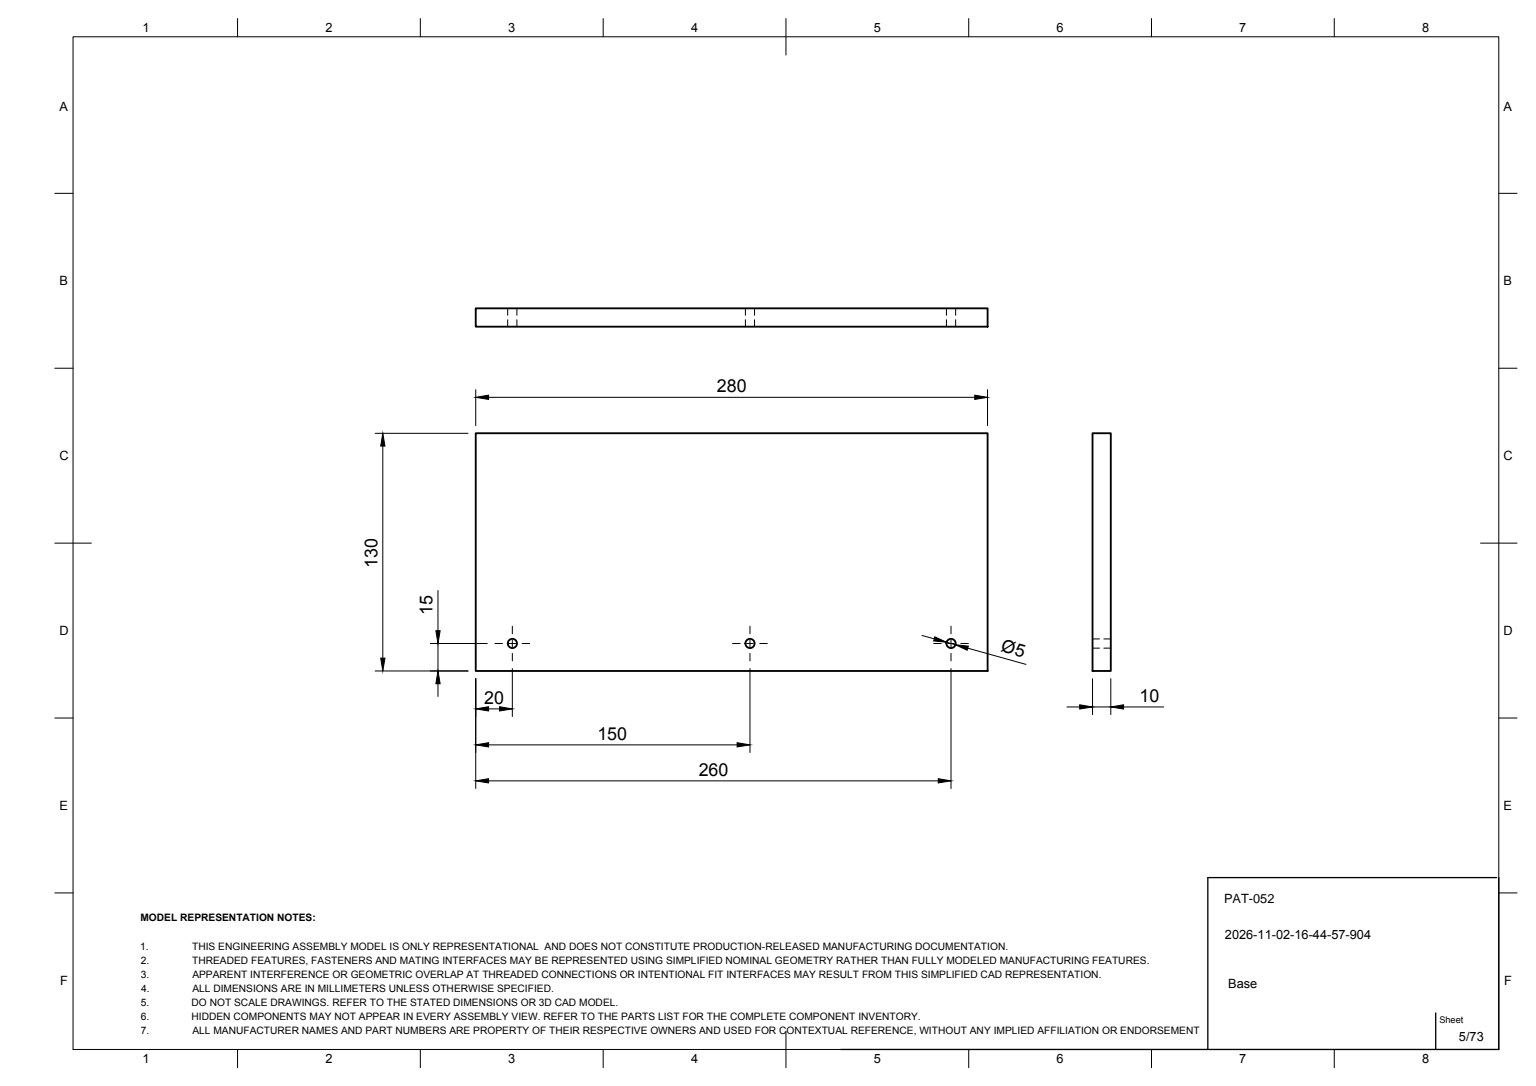
ISO-10303-21;
HEADER;
/* Generated by software containing ST-Developer
 * from STEP Tools, Inc. (www.steptools.com) 
 */

FILE_DESCRIPTION(
/* description */ ('Hand-crank gear train demonstrator'),
/* implementation_level */ '2;1');

FILE_NAME(
/* name */ 'Base.step',
/* time_stamp */ '2026-10-28T03:22:13-07:00',
/* author */ (''),
/* organization */ (''),
/* preprocessor_version */ 'ST-DEVELOPER v20.2',
/* originating_system */ 'Autodesk Translation Framework v15.17.0.0',
/* authorisation */ '');

FILE_SCHEMA (('AUTOMOTIVE_DESIGN { 1 0 10303 214 3 1 1 }'));
ENDSEC;

DATA;
#10=MECHANICAL_DESIGN_GEOMETRIC_PRESENTATION_REPRESENTATION('',(#1189),#62758);
#1061=SHAPE_REPRESENTATION_RELATIONSHIP('SRR','None',#63033,#1125);
#1125=ADVANCED_BREP_SHAPE_REPRESENTATION('',(#1268),#62687);
#1189=STYLED_ITEM('',(#63441),#1268);
#1268=MANIFOLD_SOLID_BREP('Body1',#16369);
#1342=FACE_BOUND('',#3067,.T.);
#1343=FACE_BOUND('',#3068,.T.);
#1344=FACE_BOUND('',#3069,.T.);
#1345=FACE_BOUND('',#3071,.T.);
#1346=FACE_BOUND('',#3072,.T.);
#1347=FACE_BOUND('',#3073,.T.);
#1633=PLANE('',#17170);
#1634=PLANE('',#17171);
#1635=PLANE('',#17172);
#1636=PLANE('',#17173);
#1637=PLANE('',#17174);
#1638=PLANE('',#17175);
#2123=FACE_OUTER_BOUND('',#3059,.T.);
#2124=FACE_OUTER_BOUND('',#3060,.T.);
#2125=FACE_OUTER_BOUND('',#3061,.T.);
#2126=FACE_OUTER_BOUND('',#3062,.T.);
#2127=FACE_OUTER_BOUND('',#3063,.T.);
#2128=FACE_OUTER_BOUND('',#3064,.T.);
#2129=FACE_OUTER_BOUND('',#3065,.T.);
#2130=FACE_OUTER_BOUND('',#3066,.T.);
#2131=FACE_OUTER_BOUND('',#3070,.T.);
#3059=EDGE_LOOP('',(#10835,#10836,#10837,#10838));
#3060=EDGE_LOOP('',(#10839,#10840,#10841,#10842));
#3061=EDGE_LOOP('',(#10843,#10844,#10845,#10846));
#3062=EDGE_LOOP('',(#10847,#10848,#10849,#10850));
#3063=EDGE_LOOP('',(#10851,#10852,#10853,#10854));
#3064=EDGE_LOOP('',(#10855,#10856,#10857,#10858));
#3065=EDGE_LOOP('',(#10859,#10860,#10861,#10862));
#3066=EDGE_LOOP('',(#10863,#10864,#10865,#10866));
#3067=EDGE_LOOP('',(#10867));
#3068=EDGE_LOOP('',(#10868));
#3069=EDGE_LOOP('',(#10869));
#3070=EDGE_LOOP('',(#10870,#10871,#10872,#10873));
#3071=EDGE_LOOP('',(#10874));
#3072=EDGE_LOOP('',(#10875));
#3073=EDGE_LOOP('',(#10876));
#4286=LINE('',#23316,#5418);
#4287=LINE('',#23322,#5419);
#4288=LINE('',#23328,#5420);
#4289=LINE('',#23333,#5421);
#4290=LINE('',#23335,#5422);
#4291=LINE('',#23337,#5423);
#4292=LINE('',#23338,#5424);
#4293=LINE('',#23341,#5425);
#4294=LINE('',#23343,#5426);
#4295=LINE('',#23344,#5427);
#4296=LINE('',#23347,#5428);
#4297=LINE('',#23349,#5429);
#4298=LINE('',#23350,#5430);
#4299=LINE('',#23352,#5431);
#4300=LINE('',#23353,#5432);
#5418=VECTOR('',#18841,0.25);
#5419=VECTOR('',#18848,0.25);
#5420=VECTOR('',#18855,0.25);
#5421=VECTOR('',#18860,1.);
#5422=VECTOR('',#18861,1.);
#5423=VECTOR('',#18862,1.);
#5424=VECTOR('',#18863,1.);
#5425=VECTOR('',#18866,1.);
#5426=VECTOR('',#18867,1.);
#5427=VECTOR('',#18868,1.);
#5428=VECTOR('',#18871,1.);
#5429=VECTOR('',#18872,1.);
#5430=VECTOR('',#18873,1.);
#5431=VECTOR('',#18876,1.);
#5432=VECTOR('',#18877,1.);
#6550=CIRCLE('',#17162,0.25);
#6551=CIRCLE('',#17163,0.25);
#6552=CIRCLE('',#17165,0.25);
#6553=CIRCLE('',#17166,0.25);
#6554=CIRCLE('',#17168,0.25);
#6555=CIRCLE('',#17169,0.25);
#7212=VERTEX_POINT('',#23313);
#7213=VERTEX_POINT('',#23315);
#7214=VERTEX_POINT('',#23319);
#7215=VERTEX_POINT('',#23321);
#7216=VERTEX_POINT('',#23325);
#7217=VERTEX_POINT('',#23327);
#7218=VERTEX_POINT('',#23331);
#7219=VERTEX_POINT('',#23332);
#7220=VERTEX_POINT('',#23334);
#7221=VERTEX_POINT('',#23336);
#7222=VERTEX_POINT('',#23340);
#7223=VERTEX_POINT('',#23342);
#7224=VERTEX_POINT('',#23346);
#7225=VERTEX_POINT('',#23348);
#8669=EDGE_CURVE('',#7212,#7212,#6550,.T.);
#8670=EDGE_CURVE('',#7212,#7213,#4286,.T.);
#8671=EDGE_CURVE('',#7213,#7213,#6551,.T.);
#8672=EDGE_CURVE('',#7214,#7214,#6552,.T.);
#8673=EDGE_CURVE('',#7214,#7215,#4287,.T.);
#8674=EDGE_CURVE('',#7215,#7215,#6553,.T.);
#8675=EDGE_CURVE('',#7216,#7216,#6554,.T.);
#8676=EDGE_CURVE('',#7216,#7217,#4288,.T.);
#8677=EDGE_CURVE('',#7217,#7217,#6555,.T.);
#8678=EDGE_CURVE('',#7218,#7219,#4289,.T.);
#8679=EDGE_CURVE('',#7219,#7220,#4290,.T.);
#8680=EDGE_CURVE('',#7221,#7220,#4291,.T.);
#8681=EDGE_CURVE('',#7218,#7221,#4292,.T.);
#8682=EDGE_CURVE('',#7222,#7218,#4293,.T.);
#8683=EDGE_CURVE('',#7223,#7221,#4294,.T.);
#8684=EDGE_CURVE('',#7222,#7223,#4295,.T.);
#8685=EDGE_CURVE('',#7224,#7222,#4296,.T.);
#8686=EDGE_CURVE('',#7225,#7223,#4297,.T.);
#8687=EDGE_CURVE('',#7224,#7225,#4298,.T.);
#8688=EDGE_CURVE('',#7219,#7224,#4299,.T.);
#8689=EDGE_CURVE('',#7220,#7225,#4300,.T.);
#10835=ORIENTED_EDGE('',*,*,#8669,.F.);
#10836=ORIENTED_EDGE('',*,*,#8670,.T.);
#10837=ORIENTED_EDGE('',*,*,#8671,.F.);
#10838=ORIENTED_EDGE('',*,*,#8670,.F.);
#10839=ORIENTED_EDGE('',*,*,#8672,.F.);
#10840=ORIENTED_EDGE('',*,*,#8673,.T.);
#10841=ORIENTED_EDGE('',*,*,#8674,.F.);
#10842=ORIENTED_EDGE('',*,*,#8673,.F.);
#10843=ORIENTED_EDGE('',*,*,#8675,.F.);
#10844=ORIENTED_EDGE('',*,*,#8676,.T.);
#10845=ORIENTED_EDGE('',*,*,#8677,.F.);
#10846=ORIENTED_EDGE('',*,*,#8676,.F.);
#10847=ORIENTED_EDGE('',*,*,#8678,.T.);
#10848=ORIENTED_EDGE('',*,*,#8679,.T.);
#10849=ORIENTED_EDGE('',*,*,#8680,.F.);
#10850=ORIENTED_EDGE('',*,*,#8681,.F.);
#10851=ORIENTED_EDGE('',*,*,#8682,.T.);
#10852=ORIENTED_EDGE('',*,*,#8681,.T.);
#10853=ORIENTED_EDGE('',*,*,#8683,.F.);
#10854=ORIENTED_EDGE('',*,*,#8684,.F.);
#10855=ORIENTED_EDGE('',*,*,#8685,.T.);
#10856=ORIENTED_EDGE('',*,*,#8684,.T.);
#10857=ORIENTED_EDGE('',*,*,#8686,.F.);
#10858=ORIENTED_EDGE('',*,*,#8687,.F.);
#10859=ORIENTED_EDGE('',*,*,#8688,.T.);
#10860=ORIENTED_EDGE('',*,*,#8687,.T.);
#10861=ORIENTED_EDGE('',*,*,#8689,.F.);
#10862=ORIENTED_EDGE('',*,*,#8679,.F.);
#10863=ORIENTED_EDGE('',*,*,#8689,.T.);
#10864=ORIENTED_EDGE('',*,*,#8686,.T.);
#10865=ORIENTED_EDGE('',*,*,#8683,.T.);
#10866=ORIENTED_EDGE('',*,*,#8680,.T.);
#10867=ORIENTED_EDGE('',*,*,#8671,.T.);
#10868=ORIENTED_EDGE('',*,*,#8674,.T.);
#10869=ORIENTED_EDGE('',*,*,#8677,.T.);
#10870=ORIENTED_EDGE('',*,*,#8688,.F.);
#10871=ORIENTED_EDGE('',*,*,#8678,.F.);
#10872=ORIENTED_EDGE('',*,*,#8682,.F.);
#10873=ORIENTED_EDGE('',*,*,#8685,.F.);
#10874=ORIENTED_EDGE('',*,*,#8669,.T.);
#10875=ORIENTED_EDGE('',*,*,#8672,.T.);
#10876=ORIENTED_EDGE('',*,*,#8675,.T.);
#15167=CYLINDRICAL_SURFACE('',#17161,0.25);
#15168=CYLINDRICAL_SURFACE('',#17164,0.25);
#15169=CYLINDRICAL_SURFACE('',#17167,0.25);
#15433=ADVANCED_FACE('',(#2123),#15167,.F.);
#15434=ADVANCED_FACE('',(#2124),#15168,.F.);
#15435=ADVANCED_FACE('',(#2125),#15169,.F.);
#15436=ADVANCED_FACE('',(#2126),#1633,.T.);
#15437=ADVANCED_FACE('',(#2127),#1634,.T.);
#15438=ADVANCED_FACE('',(#2128),#1635,.T.);
#15439=ADVANCED_FACE('',(#2129),#1636,.T.);
#15440=ADVANCED_FACE('',(#2130,#1342,#1343,#1344),#1637,.T.);
#15441=ADVANCED_FACE('',(#2131,#1345,#1346,#1347),#1638,.F.);
#16369=CLOSED_SHELL('',(#15433,#15434,#15435,#15436,#15437,#15438,#15439,
#15440,#15441));
#17160=AXIS2_PLACEMENT_3D('',#23311,#18835,#18836);
#17161=AXIS2_PLACEMENT_3D('',#23312,#18837,#18838);
#17162=AXIS2_PLACEMENT_3D('',#23314,#18839,#18840);
#17163=AXIS2_PLACEMENT_3D('',#23317,#18842,#18843);
#17164=AXIS2_PLACEMENT_3D('',#23318,#18844,#18845);
#17165=AXIS2_PLACEMENT_3D('',#23320,#18846,#18847);
#17166=AXIS2_PLACEMENT_3D('',#23323,#18849,#18850);
#17167=AXIS2_PLACEMENT_3D('',#23324,#18851,#18852);
#17168=AXIS2_PLACEMENT_3D('',#23326,#18853,#18854);
#17169=AXIS2_PLACEMENT_3D('',#23329,#18856,#18857);
#17170=AXIS2_PLACEMENT_3D('',#23330,#18858,#18859);
#17171=AXIS2_PLACEMENT_3D('',#23339,#18864,#18865);
#17172=AXIS2_PLACEMENT_3D('',#23345,#18869,#18870);
#17173=AXIS2_PLACEMENT_3D('',#23351,#18874,#18875);
#17174=AXIS2_PLACEMENT_3D('',#23354,#18878,#18879);
#17175=AXIS2_PLACEMENT_3D('',#23355,#18880,#18881);
#18835=DIRECTION('axis',(0.,0.,1.));
#18836=DIRECTION('refdir',(1.,0.,0.));
#18837=DIRECTION('center_axis',(0.,0.,1.));
#18838=DIRECTION('ref_axis',(1.,0.,0.));
#18839=DIRECTION('center_axis',(0.,0.,1.));
#18840=DIRECTION('ref_axis',(1.,0.,0.));
#18841=DIRECTION('',(0.,0.,1.));
#18842=DIRECTION('center_axis',(0.,0.,-1.));
#18843=DIRECTION('ref_axis',(1.,0.,0.));
#18844=DIRECTION('center_axis',(0.,0.,1.));
#18845=DIRECTION('ref_axis',(1.,0.,0.));
#18846=DIRECTION('center_axis',(0.,0.,1.));
#18847=DIRECTION('ref_axis',(1.,0.,0.));
#18848=DIRECTION('',(0.,0.,1.));
#18849=DIRECTION('center_axis',(0.,0.,-1.));
#18850=DIRECTION('ref_axis',(1.,0.,0.));
#18851=DIRECTION('center_axis',(0.,0.,1.));
#18852=DIRECTION('ref_axis',(1.,0.,0.));
#18853=DIRECTION('center_axis',(0.,0.,1.));
#18854=DIRECTION('ref_axis',(1.,0.,0.));
#18855=DIRECTION('',(0.,0.,1.));
#18856=DIRECTION('center_axis',(0.,0.,-1.));
#18857=DIRECTION('ref_axis',(1.,0.,0.));
#18858=DIRECTION('center_axis',(0.,1.,0.));
#18859=DIRECTION('ref_axis',(-1.,0.,0.));
#18860=DIRECTION('',(-1.,0.,0.));
#18861=DIRECTION('',(0.,0.,1.));
#18862=DIRECTION('',(-1.,0.,0.));
#18863=DIRECTION('',(0.,0.,1.));
#18864=DIRECTION('center_axis',(1.,0.,0.));
#18865=DIRECTION('ref_axis',(0.,1.,0.));
#18866=DIRECTION('',(0.,1.,0.));
#18867=DIRECTION('',(0.,1.,0.));
#18868=DIRECTION('',(0.,0.,1.));
#18869=DIRECTION('center_axis',(0.,-1.,0.));
#18870=DIRECTION('ref_axis',(1.,0.,0.));
#18871=DIRECTION('',(1.,0.,0.));
#18872=DIRECTION('',(1.,0.,0.));
#18873=DIRECTION('',(0.,0.,1.));
#18874=DIRECTION('center_axis',(-1.,0.,0.));
#18875=DIRECTION('ref_axis',(0.,-1.,0.));
#18876=DIRECTION('',(0.,-1.,0.));
#18877=DIRECTION('',(0.,-1.,0.));
#18878=DIRECTION('center_axis',(0.,0.,1.));
#18879=DIRECTION('ref_axis',(1.,0.,0.));
#18880=DIRECTION('center_axis',(0.,0.,1.));
#18881=DIRECTION('ref_axis',(1.,0.,0.));
#23311=CARTESIAN_POINT('',(0.,0.,0.));
#23312=CARTESIAN_POINT('Origin',(-2.,-5.,-0.1));
#23313=CARTESIAN_POINT('',(-2.25,-5.,0.));
#23314=CARTESIAN_POINT('Origin',(-2.,-5.,0.));
#23315=CARTESIAN_POINT('',(-2.25,-5.,1.));
#23316=CARTESIAN_POINT('',(-2.25,-5.,-0.1));
#23317=CARTESIAN_POINT('Origin',(-2.,-5.,1.));
#23318=CARTESIAN_POINT('Origin',(9.,-5.,-0.1));
#23319=CARTESIAN_POINT('',(8.75,-5.,0.));
#23320=CARTESIAN_POINT('Origin',(9.,-5.,0.));
#23321=CARTESIAN_POINT('',(8.75,-5.,1.));
#23322=CARTESIAN_POINT('',(8.75,-5.,-0.1));
#23323=CARTESIAN_POINT('Origin',(9.,-5.,1.));
#23324=CARTESIAN_POINT('Origin',(22.,-5.,-0.1));
#23325=CARTESIAN_POINT('',(21.75,-5.,0.));
#23326=CARTESIAN_POINT('Origin',(22.,-5.,0.));
#23327=CARTESIAN_POINT('',(21.75,-5.,1.));
#23328=CARTESIAN_POINT('',(21.75,-5.,-0.1));
#23329=CARTESIAN_POINT('Origin',(22.,-5.,1.));
#23330=CARTESIAN_POINT('Origin',(24.,6.5,0.));
#23331=CARTESIAN_POINT('',(24.,6.5,0.));
#23332=CARTESIAN_POINT('',(-4.,6.5,0.));
#23333=CARTESIAN_POINT('',(24.,6.5,0.));
#23334=CARTESIAN_POINT('',(-4.,6.5,1.));
#23335=CARTESIAN_POINT('',(-4.,6.5,0.));
#23336=CARTESIAN_POINT('',(24.,6.5,1.));
#23337=CARTESIAN_POINT('',(24.,6.5,1.));
#23338=CARTESIAN_POINT('',(24.,6.5,0.));
#23339=CARTESIAN_POINT('Origin',(24.,-6.5,0.));
#23340=CARTESIAN_POINT('',(24.,-6.5,0.));
#23341=CARTESIAN_POINT('',(24.,-6.5,0.));
#23342=CARTESIAN_POINT('',(24.,-6.5,1.));
#23343=CARTESIAN_POINT('',(24.,-6.5,1.));
#23344=CARTESIAN_POINT('',(24.,-6.5,0.));
#23345=CARTESIAN_POINT('Origin',(-4.,-6.5,0.));
#23346=CARTESIAN_POINT('',(-4.,-6.5,0.));
#23347=CARTESIAN_POINT('',(-4.,-6.5,0.));
#23348=CARTESIAN_POINT('',(-4.,-6.5,1.));
#23349=CARTESIAN_POINT('',(-4.,-6.5,1.));
#23350=CARTESIAN_POINT('',(-4.,-6.5,0.));
#23351=CARTESIAN_POINT('Origin',(-4.,6.5,0.));
#23352=CARTESIAN_POINT('',(-4.,6.5,0.));
#23353=CARTESIAN_POINT('',(-4.,6.5,1.));
#23354=CARTESIAN_POINT('Origin',(10.,0.,1.));
#23355=CARTESIAN_POINT('Origin',(10.,0.,0.));
#62613=UNCERTAINTY_MEASURE_WITH_UNIT(LENGTH_MEASURE(0.001),#62759,
'DISTANCE_ACCURACY_VALUE',
'Maximum model space distance between geometric entities at asserted c
onnectivities');
#62684=UNCERTAINTY_MEASURE_WITH_UNIT(LENGTH_MEASURE(0.001),#62759,
'DISTANCE_ACCURACY_VALUE',
'Maximum model space distance between geometric entities at asserted c
onnectivities');
#62687=(
GEOMETRIC_REPRESENTATION_CONTEXT(3)
GLOBAL_UNCERTAINTY_ASSIGNED_CONTEXT((#62613))
GLOBAL_UNIT_ASSIGNED_CONTEXT((#62759,#62761,#62762))
REPRESENTATION_CONTEXT('','3D')
);
#62758=(
GEOMETRIC_REPRESENTATION_CONTEXT(3)
GLOBAL_UNCERTAINTY_ASSIGNED_CONTEXT((#62684))
GLOBAL_UNIT_ASSIGNED_CONTEXT((#62759,#62761,#62762))
REPRESENTATION_CONTEXT('','3D')
);
#62759=(
LENGTH_UNIT()
NAMED_UNIT(*)
SI_UNIT(.CENTI.,.METRE.)
);
#62761=(
NAMED_UNIT(*)
PLANE_ANGLE_UNIT()
SI_UNIT($,.RADIAN.)
);
#62762=(
NAMED_UNIT(*)
SI_UNIT($,.STERADIAN.)
SOLID_ANGLE_UNIT()
);
#62765=SHAPE_DEFINITION_REPRESENTATION(#62838,#63033);
#62838=PRODUCT_DEFINITION_SHAPE('',$,#63107);
#63033=SHAPE_REPRESENTATION('',(#17160),#62687);
#63104=PRODUCT_DEFINITION_CONTEXT('part definition',#63325,'design');
#63107=PRODUCT_DEFINITION('Base','Base',#63180,#63104);
#63180=PRODUCT_DEFINITION_FORMATION('',$,#63329);
#63325=APPLICATION_CONTEXT(
'Core Data for Automotive Mechanical Design Process');
#63326=PRODUCT_CONTEXT('part definition',#63325,'mechanical');
#63329=PRODUCT('Base','Base','Base',(#63326));
#63435=COLOUR_RGB('Dark Blue',0.08,0.2,0.34);
#63436=FILL_AREA_STYLE_COLOUR('',#63435);
#63437=FILL_AREA_STYLE('',(#63436));
#63438=SURFACE_STYLE_FILL_AREA(#63437);
#63439=SURFACE_SIDE_STYLE('',(#63438));
#63440=SURFACE_STYLE_USAGE(.BOTH.,#63439);
#63441=PRESENTATION_STYLE_ASSIGNMENT((#63440));
ENDSEC;
END-ISO-10303-21;
